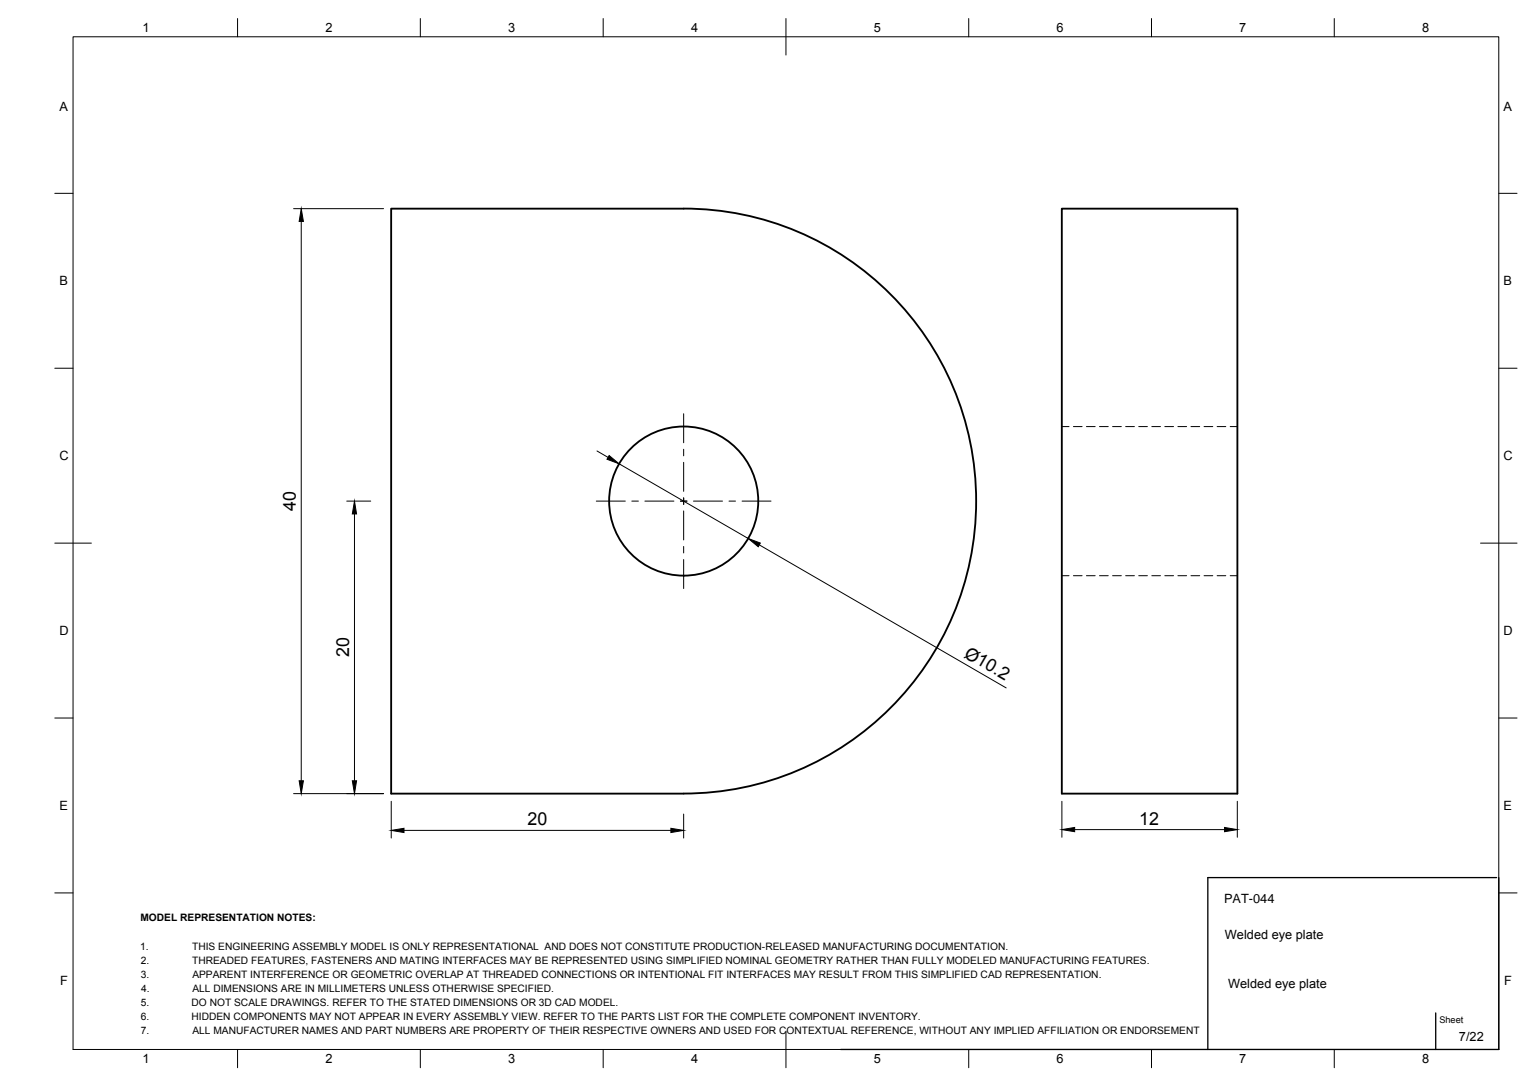
ISO-10303-21;
HEADER;
/* Generated by software containing ST-Developer
 * from STEP Tools, Inc. (www.steptools.com) 
 */

FILE_DESCRIPTION(
/* description */ ('Four-wheel beam trolley'),
/* implementation_level */ '2;1');

FILE_NAME(
/* name */ 'Welded eye plate.step',
/* time_stamp */ '2026-10-29T16:22:06-07:00',
/* author */ (''),
/* organization */ (''),
/* preprocessor_version */ 'ST-DEVELOPER v20.2',
/* originating_system */ 'Autodesk Translation Framework v15.17.0.0',
/* authorisation */ '');

FILE_SCHEMA (('AUTOMOTIVE_DESIGN { 1 0 10303 214 3 1 1 }'));
ENDSEC;

DATA;
#10=MECHANICAL_DESIGN_GEOMETRIC_PRESENTATION_REPRESENTATION('',(#280),#4777);
#246=SHAPE_REPRESENTATION_RELATIONSHIP('SRR','None',#4875,#263);
#263=ADVANCED_BREP_SHAPE_REPRESENTATION('',(#304),#4760);
#280=STYLED_ITEM('',(#5049),#304);
#304=MANIFOLD_SOLID_BREP('Body1',#2367);
#336=FACE_BOUND('',#630,.T.);
#337=FACE_BOUND('',#633,.T.);
#381=PLANE('',#2627);
#382=PLANE('',#2628);
#383=PLANE('',#2629);
#384=PLANE('',#2630);
#385=PLANE('',#2634);
#466=FACE_OUTER_BOUND('',#625,.T.);
#467=FACE_OUTER_BOUND('',#626,.T.);
#468=FACE_OUTER_BOUND('',#627,.T.);
#469=FACE_OUTER_BOUND('',#628,.T.);
#470=FACE_OUTER_BOUND('',#629,.T.);
#471=FACE_OUTER_BOUND('',#631,.T.);
#472=FACE_OUTER_BOUND('',#632,.T.);
#625=EDGE_LOOP('',(#1721,#1722,#1723,#1724));
#626=EDGE_LOOP('',(#1725,#1726,#1727,#1728));
#627=EDGE_LOOP('',(#1729,#1730,#1731,#1732));
#628=EDGE_LOOP('',(#1733,#1734,#1735,#1736));
#629=EDGE_LOOP('',(#1737,#1738,#1739,#1740));
#630=EDGE_LOOP('',(#1741));
#631=EDGE_LOOP('',(#1742,#1743,#1744,#1745));
#632=EDGE_LOOP('',(#1746,#1747,#1748,#1749));
#633=EDGE_LOOP('',(#1750));
#809=LINE('',#3874,#932);
#810=LINE('',#3879,#933);
#811=LINE('',#3881,#934);
#812=LINE('',#3883,#935);
#813=LINE('',#3884,#936);
#814=LINE('',#3888,#937);
#815=LINE('',#3890,#938);
#816=LINE('',#3892,#939);
#817=LINE('',#3893,#940);
#818=LINE('',#3895,#941);
#819=LINE('',#3896,#942);
#932=VECTOR('',#3058,0.510000000000002);
#933=VECTOR('',#3063,1.);
#934=VECTOR('',#3064,1.);
#935=VECTOR('',#3065,1.);
#936=VECTOR('',#3066,1.);
#937=VECTOR('',#3069,1.);
#938=VECTOR('',#3070,1.);
#939=VECTOR('',#3071,1.);
#940=VECTOR('',#3072,1.);
#941=VECTOR('',#3075,1.);
#942=VECTOR('',#3076,1.);
#1039=CIRCLE('',#2625,0.510000000000002);
#1040=CIRCLE('',#2626,0.510000000000002);
#1041=CIRCLE('',#2631,2.);
#1042=CIRCLE('',#2633,2.);
#1193=VERTEX_POINT('',#3871);
#1194=VERTEX_POINT('',#3873);
#1195=VERTEX_POINT('',#3877);
#1196=VERTEX_POINT('',#3878);
#1197=VERTEX_POINT('',#3880);
#1198=VERTEX_POINT('',#3882);
#1199=VERTEX_POINT('',#3886);
#1200=VERTEX_POINT('',#3887);
#1201=VERTEX_POINT('',#3889);
#1202=VERTEX_POINT('',#3891);
#1398=EDGE_CURVE('',#1193,#1193,#1039,.T.);
#1399=EDGE_CURVE('',#1193,#1194,#809,.T.);
#1400=EDGE_CURVE('',#1194,#1194,#1040,.T.);
#1401=EDGE_CURVE('',#1195,#1196,#810,.T.);
#1402=EDGE_CURVE('',#1195,#1197,#811,.T.);
#1403=EDGE_CURVE('',#1198,#1197,#812,.T.);
#1404=EDGE_CURVE('',#1196,#1198,#813,.T.);
#1405=EDGE_CURVE('',#1199,#1200,#814,.T.);
#1406=EDGE_CURVE('',#1201,#1199,#815,.T.);
#1407=EDGE_CURVE('',#1202,#1201,#816,.T.);
#1408=EDGE_CURVE('',#1200,#1202,#817,.T.);
#1409=EDGE_CURVE('',#1197,#1202,#818,.T.);
#1410=EDGE_CURVE('',#1200,#1195,#819,.T.);
#1411=EDGE_CURVE('',#1201,#1198,#1041,.T.);
#1412=EDGE_CURVE('',#1199,#1196,#1042,.T.);
#1721=ORIENTED_EDGE('',*,*,#1398,.F.);
#1722=ORIENTED_EDGE('',*,*,#1399,.T.);
#1723=ORIENTED_EDGE('',*,*,#1400,.F.);
#1724=ORIENTED_EDGE('',*,*,#1399,.F.);
#1725=ORIENTED_EDGE('',*,*,#1401,.F.);
#1726=ORIENTED_EDGE('',*,*,#1402,.T.);
#1727=ORIENTED_EDGE('',*,*,#1403,.F.);
#1728=ORIENTED_EDGE('',*,*,#1404,.F.);
#1729=ORIENTED_EDGE('',*,*,#1405,.F.);
#1730=ORIENTED_EDGE('',*,*,#1406,.F.);
#1731=ORIENTED_EDGE('',*,*,#1407,.F.);
#1732=ORIENTED_EDGE('',*,*,#1408,.F.);
#1733=ORIENTED_EDGE('',*,*,#1409,.F.);
#1734=ORIENTED_EDGE('',*,*,#1402,.F.);
#1735=ORIENTED_EDGE('',*,*,#1410,.F.);
#1736=ORIENTED_EDGE('',*,*,#1408,.T.);
#1737=ORIENTED_EDGE('',*,*,#1411,.T.);
#1738=ORIENTED_EDGE('',*,*,#1403,.T.);
#1739=ORIENTED_EDGE('',*,*,#1409,.T.);
#1740=ORIENTED_EDGE('',*,*,#1407,.T.);
#1741=ORIENTED_EDGE('',*,*,#1400,.T.);
#1742=ORIENTED_EDGE('',*,*,#1404,.T.);
#1743=ORIENTED_EDGE('',*,*,#1411,.F.);
#1744=ORIENTED_EDGE('',*,*,#1406,.T.);
#1745=ORIENTED_EDGE('',*,*,#1412,.T.);
#1746=ORIENTED_EDGE('',*,*,#1412,.F.);
#1747=ORIENTED_EDGE('',*,*,#1405,.T.);
#1748=ORIENTED_EDGE('',*,*,#1410,.T.);
#1749=ORIENTED_EDGE('',*,*,#1401,.T.);
#1750=ORIENTED_EDGE('',*,*,#1398,.T.);
#2183=CYLINDRICAL_SURFACE('',#2624,0.510000000000002);
#2184=CYLINDRICAL_SURFACE('',#2632,2.);
#2242=ADVANCED_FACE('',(#466),#2183,.F.);
#2243=ADVANCED_FACE('',(#467),#381,.T.);
#2244=ADVANCED_FACE('',(#468),#382,.T.);
#2245=ADVANCED_FACE('',(#469),#383,.T.);
#2246=ADVANCED_FACE('',(#470,#336),#384,.T.);
#2247=ADVANCED_FACE('',(#471),#2184,.T.);
#2248=ADVANCED_FACE('',(#472,#337),#385,.F.);
#2367=CLOSED_SHELL('',(#2242,#2243,#2244,#2245,#2246,#2247,#2248));
#2623=AXIS2_PLACEMENT_3D('',#3869,#3052,#3053);
#2624=AXIS2_PLACEMENT_3D('',#3870,#3054,#3055);
#2625=AXIS2_PLACEMENT_3D('',#3872,#3056,#3057);
#2626=AXIS2_PLACEMENT_3D('',#3875,#3059,#3060);
#2627=AXIS2_PLACEMENT_3D('',#3876,#3061,#3062);
#2628=AXIS2_PLACEMENT_3D('',#3885,#3067,#3068);
#2629=AXIS2_PLACEMENT_3D('',#3894,#3073,#3074);
#2630=AXIS2_PLACEMENT_3D('',#3897,#3077,#3078);
#2631=AXIS2_PLACEMENT_3D('',#3898,#3079,#3080);
#2632=AXIS2_PLACEMENT_3D('',#3899,#3081,#3082);
#2633=AXIS2_PLACEMENT_3D('',#3900,#3083,#3084);
#2634=AXIS2_PLACEMENT_3D('',#3901,#3085,#3086);
#3052=DIRECTION('axis',(0.,0.,1.));
#3053=DIRECTION('refdir',(1.,0.,0.));
#3054=DIRECTION('center_axis',(0.,1.,0.));
#3055=DIRECTION('ref_axis',(1.,0.,0.));
#3056=DIRECTION('center_axis',(0.,1.,0.));
#3057=DIRECTION('ref_axis',(1.,0.,0.));
#3058=DIRECTION('',(0.,1.,0.));
#3059=DIRECTION('center_axis',(0.,-1.,0.));
#3060=DIRECTION('ref_axis',(1.,0.,0.));
#3061=DIRECTION('center_axis',(-1.,0.,0.));
#3062=DIRECTION('ref_axis',(0.,0.,1.));
#3063=DIRECTION('',(0.,0.,-1.));
#3064=DIRECTION('',(0.,1.,0.));
#3065=DIRECTION('',(0.,0.,1.));
#3066=DIRECTION('',(0.,1.,0.));
#3067=DIRECTION('center_axis',(1.,0.,0.));
#3068=DIRECTION('ref_axis',(0.,0.,-1.));
#3069=DIRECTION('',(0.,0.,1.));
#3070=DIRECTION('',(0.,-1.,0.));
#3071=DIRECTION('',(0.,0.,-1.));
#3072=DIRECTION('',(0.,1.,0.));
#3073=DIRECTION('center_axis',(0.,0.,1.));
#3074=DIRECTION('ref_axis',(1.,0.,0.));
#3075=DIRECTION('',(1.,0.,0.));
#3076=DIRECTION('',(-1.,0.,0.));
#3077=DIRECTION('center_axis',(0.,1.,0.));
#3078=DIRECTION('ref_axis',(1.,0.,0.));
#3079=DIRECTION('center_axis',(0.,1.,0.));
#3080=DIRECTION('ref_axis',(1.,0.,0.));
#3081=DIRECTION('center_axis',(0.,1.,0.));
#3082=DIRECTION('ref_axis',(1.,0.,0.));
#3083=DIRECTION('center_axis',(0.,1.,0.));
#3084=DIRECTION('ref_axis',(1.,0.,0.));
#3085=DIRECTION('center_axis',(0.,1.,0.));
#3086=DIRECTION('ref_axis',(1.,0.,0.));
#3869=CARTESIAN_POINT('',(0.,0.,0.));
#3870=CARTESIAN_POINT('Origin',(-21.,-0.7,-2.));
#3871=CARTESIAN_POINT('',(-21.51,-0.6,-2.));
#3872=CARTESIAN_POINT('Origin',(-21.,-0.6,-2.));
#3873=CARTESIAN_POINT('',(-21.51,0.6,-2.));
#3874=CARTESIAN_POINT('',(-21.51,-0.7,-2.));
#3875=CARTESIAN_POINT('Origin',(-21.,0.6,-2.));
#3876=CARTESIAN_POINT('Origin',(-23.,-0.6,-2.));
#3877=CARTESIAN_POINT('',(-23.,-0.6,0.));
#3878=CARTESIAN_POINT('',(-23.,-0.6,-2.));
#3879=CARTESIAN_POINT('',(-23.,-0.6,0.));
#3880=CARTESIAN_POINT('',(-23.,0.6,0.));
#3881=CARTESIAN_POINT('',(-23.,-0.6,0.));
#3882=CARTESIAN_POINT('',(-23.,0.6,-2.));
#3883=CARTESIAN_POINT('',(-23.,0.6,0.));
#3884=CARTESIAN_POINT('',(-23.,-0.6,-2.));
#3885=CARTESIAN_POINT('Origin',(-19.,-0.6,0.));
#3886=CARTESIAN_POINT('',(-19.,-0.6,-2.));
#3887=CARTESIAN_POINT('',(-19.,-0.6,0.));
#3888=CARTESIAN_POINT('',(-19.,-0.6,-2.));
#3889=CARTESIAN_POINT('',(-19.,0.6,-2.));
#3890=CARTESIAN_POINT('',(-19.,-0.6,-2.));
#3891=CARTESIAN_POINT('',(-19.,0.6,0.));
#3892=CARTESIAN_POINT('',(-19.,0.6,-2.));
#3893=CARTESIAN_POINT('',(-19.,-0.6,0.));
#3894=CARTESIAN_POINT('Origin',(-23.,-0.6,0.));
#3895=CARTESIAN_POINT('',(-19.,0.6,0.));
#3896=CARTESIAN_POINT('',(-19.,-0.6,0.));
#3897=CARTESIAN_POINT('Origin',(-21.,0.6,-2.));
#3898=CARTESIAN_POINT('Origin',(-21.,0.6,-2.));
#3899=CARTESIAN_POINT('Origin',(-21.,-0.6,-2.));
#3900=CARTESIAN_POINT('Origin',(-21.,-0.6,-2.));
#3901=CARTESIAN_POINT('Origin',(-21.,-0.6,-2.));
#4738=UNCERTAINTY_MEASURE_WITH_UNIT(LENGTH_MEASURE(0.001),#4778,
'DISTANCE_ACCURACY_VALUE',
'Maximum model space distance between geometric entities at asserted c
onnectivities');
#4755=UNCERTAINTY_MEASURE_WITH_UNIT(LENGTH_MEASURE(0.001),#4778,
'DISTANCE_ACCURACY_VALUE',
'Maximum model space distance between geometric entities at asserted c
onnectivities');
#4760=(
GEOMETRIC_REPRESENTATION_CONTEXT(3)
GLOBAL_UNCERTAINTY_ASSIGNED_CONTEXT((#4738))
GLOBAL_UNIT_ASSIGNED_CONTEXT((#4778,#4780,#4781))
REPRESENTATION_CONTEXT('','3D')
);
#4777=(
GEOMETRIC_REPRESENTATION_CONTEXT(3)
GLOBAL_UNCERTAINTY_ASSIGNED_CONTEXT((#4755))
GLOBAL_UNIT_ASSIGNED_CONTEXT((#4778,#4780,#4781))
REPRESENTATION_CONTEXT('','3D')
);
#4778=(
LENGTH_UNIT()
NAMED_UNIT(*)
SI_UNIT(.CENTI.,.METRE.)
);
#4780=(
NAMED_UNIT(*)
PLANE_ANGLE_UNIT()
SI_UNIT($,.RADIAN.)
);
#4781=(
NAMED_UNIT(*)
SI_UNIT($,.STERADIAN.)
SOLID_ANGLE_UNIT()
);
#4786=SHAPE_DEFINITION_REPRESENTATION(#4807,#4875);
#4807=PRODUCT_DEFINITION_SHAPE('',$,#4897);
#4875=SHAPE_REPRESENTATION('',(#2623),#4760);
#4892=PRODUCT_DEFINITION_CONTEXT('part definition',#4957,'design');
#4897=PRODUCT_DEFINITION('Welded eye plate','Welded eye plate',#4918,#4892);
#4918=PRODUCT_DEFINITION_FORMATION('',$,#4963);
#4957=APPLICATION_CONTEXT(
'Core Data for Automotive Mechanical Design Process');
#4958=PRODUCT_CONTEXT('part definition',#4957,'mechanical');
#4963=PRODUCT('Welded eye plate','Welded eye plate','Welded eye plate',
(#4958));
#5043=COLOUR_RGB('Sky Blue',0.24,0.69,0.87);
#5044=FILL_AREA_STYLE_COLOUR('',#5043);
#5045=FILL_AREA_STYLE('',(#5044));
#5046=SURFACE_STYLE_FILL_AREA(#5045);
#5047=SURFACE_SIDE_STYLE('',(#5046));
#5048=SURFACE_STYLE_USAGE(.BOTH.,#5047);
#5049=PRESENTATION_STYLE_ASSIGNMENT((#5048));
ENDSEC;
END-ISO-10303-21;
